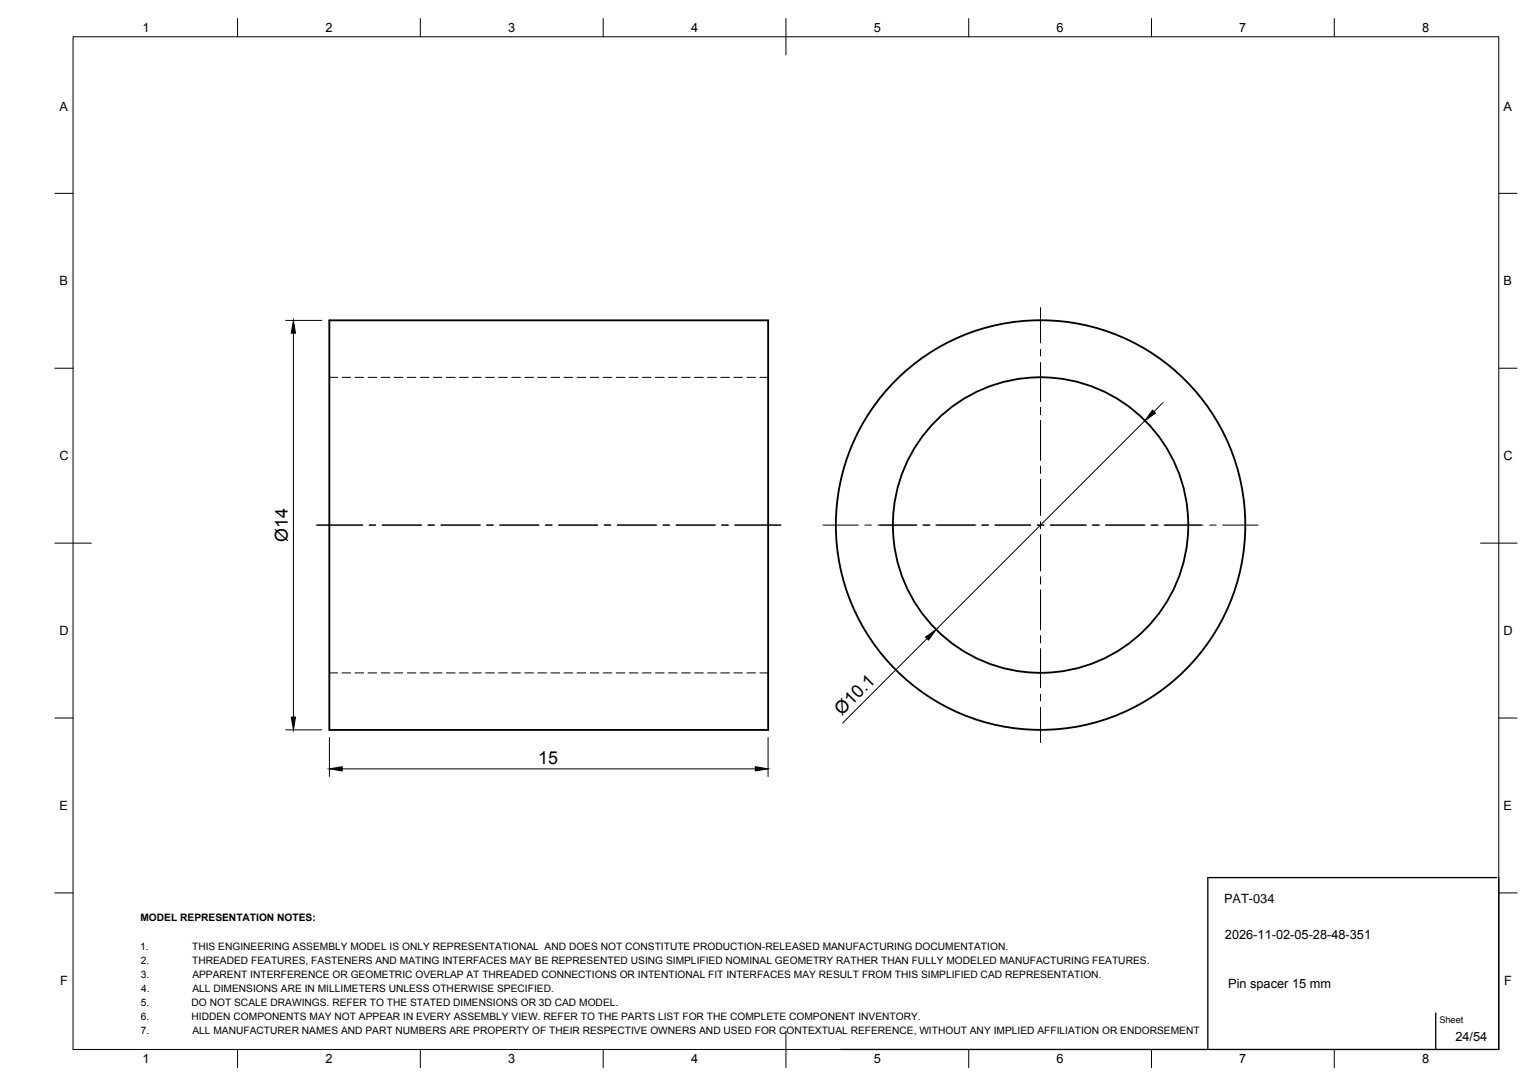
ISO-10303-21;
HEADER;
/* Generated by software containing ST-Developer
 * from STEP Tools, Inc. (www.steptools.com) 
 */

FILE_DESCRIPTION(
/* description */ ('Fatigue rig crank-slider'),
/* implementation_level */ '2;1');

FILE_NAME(
/* name */ 'Pin spacer 15 mm.step',
/* time_stamp */ '2026-10-28T03:24:50-07:00',
/* author */ (''),
/* organization */ (''),
/* preprocessor_version */ 'ST-DEVELOPER v20.2',
/* originating_system */ 'Autodesk Translation Framework v15.17.0.0',
/* authorisation */ '');

FILE_SCHEMA (('AUTOMOTIVE_DESIGN { 1 0 10303 214 3 1 1 }'));
ENDSEC;

DATA;
#10=MECHANICAL_DESIGN_GEOMETRIC_PRESENTATION_REPRESENTATION('',(#610),#16911);
#509=SHAPE_REPRESENTATION_RELATIONSHIP('SRR','None',#17150,#559);
#559=ADVANCED_BREP_SHAPE_REPRESENTATION('',(#667),#16879);
#610=STYLED_ITEM('',(#17487),#667);
#667=MANIFOLD_SOLID_BREP('Body1',#8903);
#835=FACE_BOUND('',#2145,.T.);
#836=FACE_BOUND('',#2147,.T.);
#1057=PLANE('',#10004);
#1058=PLANE('',#10005);
#1484=FACE_OUTER_BOUND('',#2142,.T.);
#1485=FACE_OUTER_BOUND('',#2143,.T.);
#1486=FACE_OUTER_BOUND('',#2144,.T.);
#1487=FACE_OUTER_BOUND('',#2146,.T.);
#2142=EDGE_LOOP('',(#7122,#7123,#7124,#7125));
#2143=EDGE_LOOP('',(#7126,#7127,#7128,#7129));
#2144=EDGE_LOOP('',(#7130));
#2145=EDGE_LOOP('',(#7131));
#2146=EDGE_LOOP('',(#7132));
#2147=EDGE_LOOP('',(#7133));
#2778=LINE('',#15183,#3424);
#2779=LINE('',#15189,#3425);
#3424=VECTOR('',#11898,0.505);
#3425=VECTOR('',#11905,0.7);
#3961=CIRCLE('',#9999,0.505);
#3962=CIRCLE('',#10000,0.505);
#3963=CIRCLE('',#10002,0.7);
#3964=CIRCLE('',#10003,0.7);
#4533=VERTEX_POINT('',#15180);
#4534=VERTEX_POINT('',#15182);
#4535=VERTEX_POINT('',#15186);
#4536=VERTEX_POINT('',#15188);
#5459=EDGE_CURVE('',#4533,#4533,#3961,.T.);
#5460=EDGE_CURVE('',#4533,#4534,#2778,.T.);
#5461=EDGE_CURVE('',#4534,#4534,#3962,.T.);
#5462=EDGE_CURVE('',#4535,#4535,#3963,.T.);
#5463=EDGE_CURVE('',#4535,#4536,#2779,.T.);
#5464=EDGE_CURVE('',#4536,#4536,#3964,.T.);
#7122=ORIENTED_EDGE('',*,*,#5459,.F.);
#7123=ORIENTED_EDGE('',*,*,#5460,.T.);
#7124=ORIENTED_EDGE('',*,*,#5461,.T.);
#7125=ORIENTED_EDGE('',*,*,#5460,.F.);
#7126=ORIENTED_EDGE('',*,*,#5462,.F.);
#7127=ORIENTED_EDGE('',*,*,#5463,.T.);
#7128=ORIENTED_EDGE('',*,*,#5464,.T.);
#7129=ORIENTED_EDGE('',*,*,#5463,.F.);
#7130=ORIENTED_EDGE('',*,*,#5462,.T.);
#7131=ORIENTED_EDGE('',*,*,#5459,.T.);
#7132=ORIENTED_EDGE('',*,*,#5464,.F.);
#7133=ORIENTED_EDGE('',*,*,#5461,.F.);
#8294=CYLINDRICAL_SURFACE('',#9998,0.505);
#8295=CYLINDRICAL_SURFACE('',#10001,0.7);
#8622=ADVANCED_FACE('',(#1484),#8294,.F.);
#8623=ADVANCED_FACE('',(#1485),#8295,.T.);
#8624=ADVANCED_FACE('',(#1486,#835),#1057,.T.);
#8625=ADVANCED_FACE('',(#1487,#836),#1058,.F.);
#8903=CLOSED_SHELL('',(#8622,#8623,#8624,#8625));
#9997=AXIS2_PLACEMENT_3D('',#15178,#11892,#11893);
#9998=AXIS2_PLACEMENT_3D('',#15179,#11894,#11895);
#9999=AXIS2_PLACEMENT_3D('',#15181,#11896,#11897);
#10000=AXIS2_PLACEMENT_3D('',#15184,#11899,#11900);
#10001=AXIS2_PLACEMENT_3D('',#15185,#11901,#11902);
#10002=AXIS2_PLACEMENT_3D('',#15187,#11903,#11904);
#10003=AXIS2_PLACEMENT_3D('',#15190,#11906,#11907);
#10004=AXIS2_PLACEMENT_3D('',#15191,#11908,#11909);
#10005=AXIS2_PLACEMENT_3D('',#15192,#11910,#11911);
#11892=DIRECTION('axis',(0.,0.,1.));
#11893=DIRECTION('refdir',(1.,0.,0.));
#11894=DIRECTION('center_axis',(0.,1.,0.));
#11895=DIRECTION('ref_axis',(1.,0.,0.));
#11896=DIRECTION('center_axis',(0.,-1.,0.));
#11897=DIRECTION('ref_axis',(1.,0.,0.));
#11898=DIRECTION('',(0.,-1.,0.));
#11899=DIRECTION('center_axis',(0.,-1.,0.));
#11900=DIRECTION('ref_axis',(1.,0.,0.));
#11901=DIRECTION('center_axis',(0.,1.,0.));
#11902=DIRECTION('ref_axis',(1.,0.,0.));
#11903=DIRECTION('center_axis',(0.,1.,0.));
#11904=DIRECTION('ref_axis',(1.,0.,0.));
#11905=DIRECTION('',(0.,-1.,0.));
#11906=DIRECTION('center_axis',(0.,1.,0.));
#11907=DIRECTION('ref_axis',(1.,0.,0.));
#11908=DIRECTION('center_axis',(0.,1.,0.));
#11909=DIRECTION('ref_axis',(1.,0.,0.));
#11910=DIRECTION('center_axis',(0.,1.,0.));
#11911=DIRECTION('ref_axis',(1.,0.,0.));
#15178=CARTESIAN_POINT('',(0.,0.,0.));
#15179=CARTESIAN_POINT('Origin',(1.,2.,12.));
#15180=CARTESIAN_POINT('',(0.495,3.5,12.));
#15181=CARTESIAN_POINT('Origin',(1.,3.5,12.));
#15182=CARTESIAN_POINT('',(0.495,2.,12.));
#15183=CARTESIAN_POINT('',(0.495,2.,12.));
#15184=CARTESIAN_POINT('Origin',(1.,2.,12.));
#15185=CARTESIAN_POINT('Origin',(1.,2.,12.));
#15186=CARTESIAN_POINT('',(0.3,3.5,12.));
#15187=CARTESIAN_POINT('Origin',(1.,3.5,12.));
#15188=CARTESIAN_POINT('',(0.3,2.,12.));
#15189=CARTESIAN_POINT('',(0.3,2.,12.));
#15190=CARTESIAN_POINT('Origin',(1.,2.,12.));
#15191=CARTESIAN_POINT('Origin',(1.,3.5,12.));
#15192=CARTESIAN_POINT('Origin',(1.,2.,12.));
#16820=UNCERTAINTY_MEASURE_WITH_UNIT(LENGTH_MEASURE(0.001),#16912,
'DISTANCE_ACCURACY_VALUE',
'Maximum model space distance between geometric entities at asserted c
onnectivities');
#16852=UNCERTAINTY_MEASURE_WITH_UNIT(LENGTH_MEASURE(0.001),#16912,
'DISTANCE_ACCURACY_VALUE',
'Maximum model space distance between geometric entities at asserted c
onnectivities');
#16879=(
GEOMETRIC_REPRESENTATION_CONTEXT(3)
GLOBAL_UNCERTAINTY_ASSIGNED_CONTEXT((#16820))
GLOBAL_UNIT_ASSIGNED_CONTEXT((#16912,#16914,#16915))
REPRESENTATION_CONTEXT('','3D')
);
#16911=(
GEOMETRIC_REPRESENTATION_CONTEXT(3)
GLOBAL_UNCERTAINTY_ASSIGNED_CONTEXT((#16852))
GLOBAL_UNIT_ASSIGNED_CONTEXT((#16912,#16914,#16915))
REPRESENTATION_CONTEXT('','3D')
);
#16912=(
LENGTH_UNIT()
NAMED_UNIT(*)
SI_UNIT(.CENTI.,.METRE.)
);
#16914=(
NAMED_UNIT(*)
PLANE_ANGLE_UNIT()
SI_UNIT($,.RADIAN.)
);
#16915=(
NAMED_UNIT(*)
SI_UNIT($,.STERADIAN.)
SOLID_ANGLE_UNIT()
);
#16942=SHAPE_DEFINITION_REPRESENTATION(#17002,#17150);
#17002=PRODUCT_DEFINITION_SHAPE('',$,#17209);
#17150=SHAPE_REPRESENTATION('',(#9997),#16879);
#17182=PRODUCT_DEFINITION_CONTEXT('part definition',#17358,'design');
#17209=PRODUCT_DEFINITION('Pin spacer 15 mm','Pin spacer 15 mm',#17267,
#17182);
#17267=PRODUCT_DEFINITION_FORMATION('',$,#17386);
#17358=APPLICATION_CONTEXT(
'Core Data for Automotive Mechanical Design Process');
#17359=PRODUCT_CONTEXT('part definition',#17358,'mechanical');
#17386=PRODUCT('Pin spacer 15 mm','Pin spacer 15 mm','Pin spacer 15 mm',
(#17359));
#17481=COLOUR_RGB('Grey',0.48,0.52,0.57);
#17482=FILL_AREA_STYLE_COLOUR('',#17481);
#17483=FILL_AREA_STYLE('',(#17482));
#17484=SURFACE_STYLE_FILL_AREA(#17483);
#17485=SURFACE_SIDE_STYLE('',(#17484));
#17486=SURFACE_STYLE_USAGE(.BOTH.,#17485);
#17487=PRESENTATION_STYLE_ASSIGNMENT((#17486));
ENDSEC;
END-ISO-10303-21;
